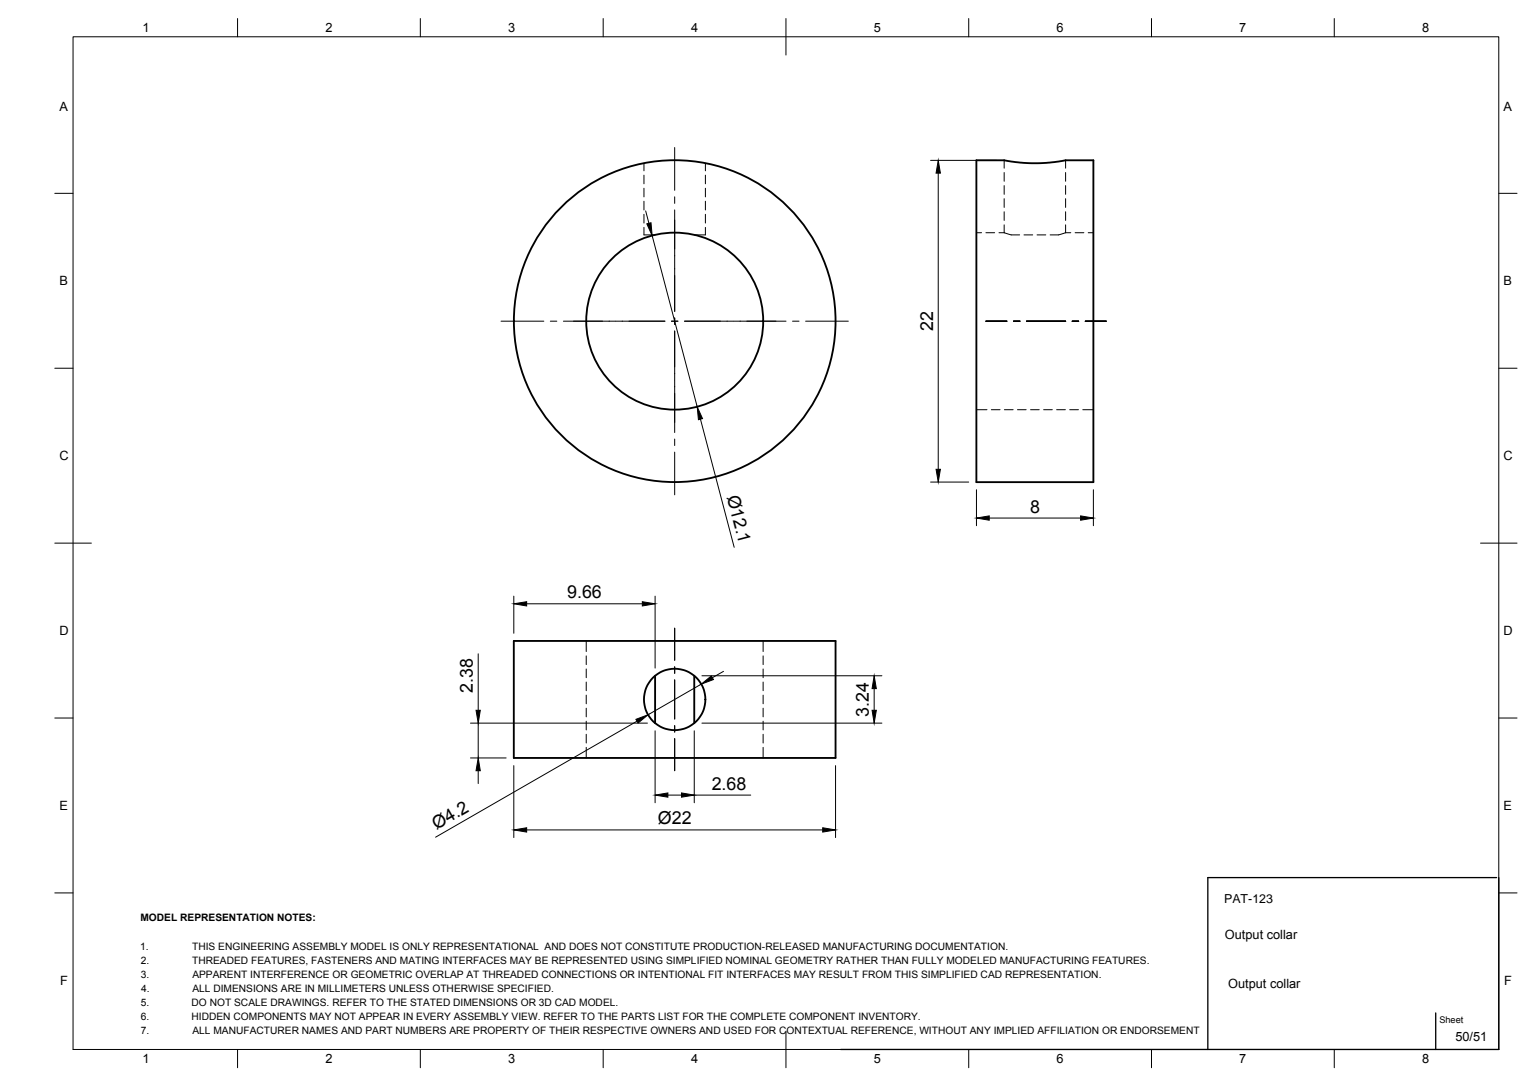
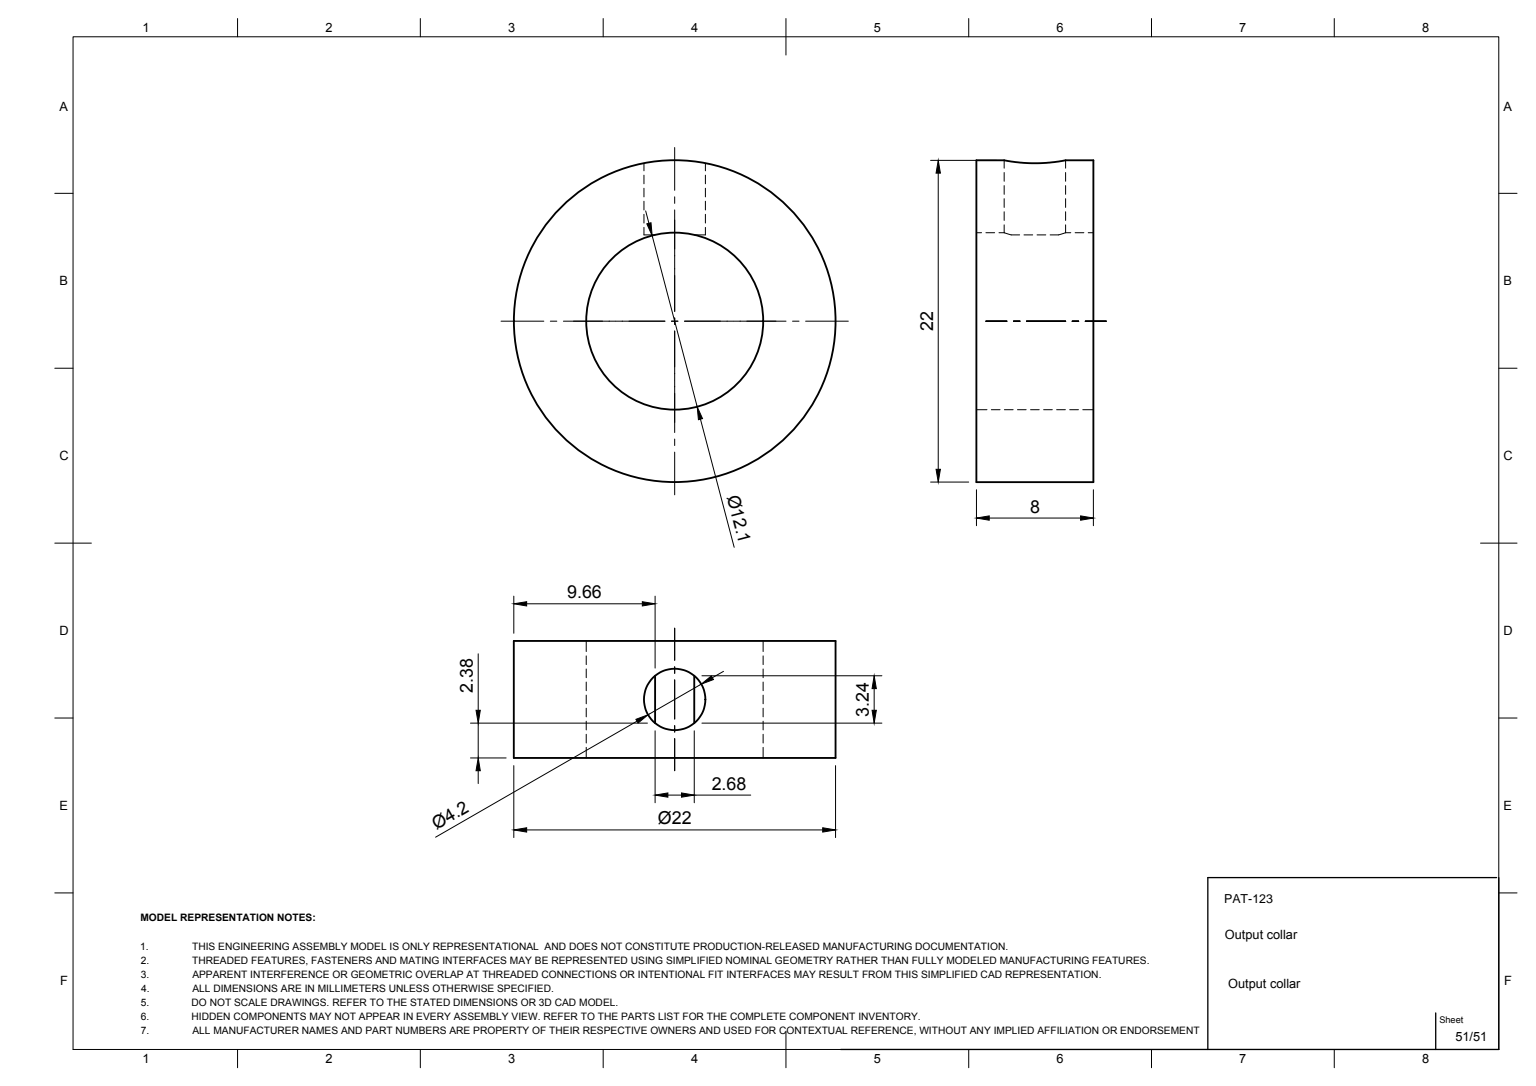
ISO-10303-21;
HEADER;
/* Generated by software containing ST-Developer
 * from STEP Tools, Inc. (www.steptools.com) 
 */

FILE_DESCRIPTION(
/* description */ ('Worm-less right-angle friction wheel drive'),
/* implementation_level */ '2;1');

FILE_NAME(
/* name */ 'Output collar.step',
/* time_stamp */ '2026-10-28T03:22:36-07:00',
/* author */ (''),
/* organization */ (''),
/* preprocessor_version */ 'ST-DEVELOPER v20.2',
/* originating_system */ 'Autodesk Translation Framework v15.17.0.0',
/* authorisation */ '');

FILE_SCHEMA (('AUTOMOTIVE_DESIGN { 1 0 10303 214 3 1 1 }'));
ENDSEC;

DATA;
#10=MECHANICAL_DESIGN_GEOMETRIC_PRESENTATION_REPRESENTATION('',(#661),#17046);
#501=B_SPLINE_CURVE_WITH_KNOTS('',3,(#16636,#16637,#16638,#16639,#16640,
#16641),.UNSPECIFIED.,.F.,.F.,(4,2,4),(0.818088904349169,0.878131747417164,
0.957937926194035),.UNSPECIFIED.);
#502=B_SPLINE_CURVE_WITH_KNOTS('',3,(#16645,#16646,#16647,#16648,#16649,
#16650),.UNSPECIFIED.,.F.,.F.,(4,2,4),(0.319312642064678,0.399118820841549,
0.459161663909543),.UNSPECIFIED.);
#503=B_SPLINE_CURVE_WITH_KNOTS('',3,(#16651,#16652,#16653,#16654,#16655,
#16656),.UNSPECIFIED.,.F.,.F.,(4,2,4),(0.179463620219813,0.239506463287807,
0.319312642064678),.UNSPECIFIED.);
#504=B_SPLINE_CURVE_WITH_KNOTS('',3,(#16657,#16658,#16659,#16660,#16661,
#16662),.UNSPECIFIED.,.F.,.F.,(4,2,4),(0.957937926194035,1.03774410497091,
1.0977869480389),.UNSPECIFIED.);
#505=B_SPLINE_CURVE_WITH_KNOTS('',3,(#16666,#16667,#16668,#16669,#16670,
#16671,#16672,#16673,#16674,#16675),.UNSPECIFIED.,.F.,.F.,(4,2,2,2,4),(0.,
0.0793157643915217,0.158631528783043,0.237943615933649,0.317255703084255),
 .UNSPECIFIED.);
#506=B_SPLINE_CURVE_WITH_KNOTS('',3,(#16677,#16678,#16679,#16680,#16681,
#16682,#16683,#16684,#16685,#16686),.UNSPECIFIED.,.F.,.F.,(4,2,2,2,4),(0.951767109252766,
1.03107919640337,1.11039128355398,1.1897070479455,1.26902281233702),
 .UNSPECIFIED.);
#507=B_SPLINE_CURVE_WITH_KNOTS('',3,(#16687,#16688,#16689,#16690,#16691,
#16692,#16693,#16694,#16695,#16696,#16697,#16698,#16699,#16700,#16701,#16702,
#16703,#16704),.UNSPECIFIED.,.F.,.F.,(4,2,2,2,2,2,2,2,4),(0.317255703084255,
0.396567790234861,0.475879877385467,0.555195641776989,0.63451140616851,
0.713827170560032,0.793142934951554,0.87245502210216,0.951767109252766),
 .UNSPECIFIED.);
#560=SHAPE_REPRESENTATION_RELATIONSHIP('SRR','None',#17306,#607);
#607=ADVANCED_BREP_SHAPE_REPRESENTATION('',(#711),#17042);
#661=STYLED_ITEM('',(#17605),#711);
#711=MANIFOLD_SOLID_BREP('Body1',#8220);
#947=FACE_BOUND('',#2343,.T.);
#948=FACE_BOUND('',#2345,.T.);
#1181=PLANE('',#9699);
#1182=PLANE('',#9703);
#1183=PLANE('',#9710);
#1184=PLANE('',#9711);
#1639=FACE_OUTER_BOUND('',#2337,.T.);
#1640=FACE_OUTER_BOUND('',#2338,.T.);
#1641=FACE_OUTER_BOUND('',#2339,.T.);
#1642=FACE_OUTER_BOUND('',#2340,.T.);
#1643=FACE_OUTER_BOUND('',#2341,.T.);
#1644=FACE_OUTER_BOUND('',#2342,.T.);
#1645=FACE_OUTER_BOUND('',#2344,.T.);
#2337=EDGE_LOOP('',(#7356,#7357));
#2338=EDGE_LOOP('',(#7358,#7359,#7360,#7361,#7362,#7363,#7364,#7365,#7366,
#7367,#7368));
#2339=EDGE_LOOP('',(#7369,#7370));
#2340=EDGE_LOOP('',(#7371,#7372,#7373,#7374,#7375,#7376,#7377,#7378,#7379,
#7380,#7381,#7382));
#2341=EDGE_LOOP('',(#7383,#7384,#7385,#7386,#7387,#7388,#7389,#7390,#7391));
#2342=EDGE_LOOP('',(#7392));
#2343=EDGE_LOOP('',(#7393));
#2344=EDGE_LOOP('',(#7394));
#2345=EDGE_LOOP('',(#7395));
#2859=LINE('',#16631,#3399);
#2860=LINE('',#16664,#3400);
#2861=LINE('',#16706,#3401);
#2862=LINE('',#16710,#3402);
#2863=LINE('',#16712,#3403);
#2864=LINE('',#16717,#3404);
#2865=LINE('',#16719,#3405);
#3399=VECTOR('',#12171,1.);
#3400=VECTOR('',#12178,0.21);
#3401=VECTOR('',#12181,1.);
#3402=VECTOR('',#12186,0.605);
#3403=VECTOR('',#12187,0.605);
#3404=VECTOR('',#12194,1.1);
#3405=VECTOR('',#12195,1.1);
#3854=CIRCLE('',#9700,0.21);
#3855=CIRCLE('',#9702,0.21);
#3856=CIRCLE('',#9705,0.605);
#3857=CIRCLE('',#9706,0.605);
#3858=CIRCLE('',#9708,1.1);
#3859=CIRCLE('',#9709,1.1);
#4479=VERTEX_POINT('',#16629);
#4480=VERTEX_POINT('',#16630);
#4481=VERTEX_POINT('',#16634);
#4482=VERTEX_POINT('',#16635);
#4483=VERTEX_POINT('',#16642);
#4484=VERTEX_POINT('',#16644);
#4485=VERTEX_POINT('',#16663);
#4486=VERTEX_POINT('',#16665);
#4487=VERTEX_POINT('',#16676);
#4488=VERTEX_POINT('',#16708);
#4489=VERTEX_POINT('',#16711);
#4490=VERTEX_POINT('',#16715);
#4491=VERTEX_POINT('',#16718);
#5447=EDGE_CURVE('',#4479,#4480,#2859,.T.);
#5448=EDGE_CURVE('',#4479,#4480,#3854,.T.);
#5449=EDGE_CURVE('',#4481,#4482,#501,.T.);
#5450=EDGE_CURVE('',#4483,#4481,#3855,.T.);
#5451=EDGE_CURVE('',#4484,#4483,#502,.T.);
#5452=EDGE_CURVE('',#4480,#4484,#503,.T.);
#5453=EDGE_CURVE('',#4482,#4479,#504,.T.);
#5454=EDGE_CURVE('',#4482,#4485,#2860,.T.);
#5455=EDGE_CURVE('',#4486,#4485,#505,.T.);
#5456=EDGE_CURVE('',#4487,#4486,#506,.T.);
#5457=EDGE_CURVE('',#4485,#4487,#507,.T.);
#5458=EDGE_CURVE('',#4483,#4481,#2861,.T.);
#5459=EDGE_CURVE('',#4488,#4488,#3856,.T.);
#5460=EDGE_CURVE('',#4488,#4484,#2862,.T.);
#5461=EDGE_CURVE('',#4482,#4489,#2863,.T.);
#5462=EDGE_CURVE('',#4489,#4489,#3857,.T.);
#5463=EDGE_CURVE('',#4490,#4490,#3858,.T.);
#5464=EDGE_CURVE('',#4490,#4487,#2864,.T.);
#5465=EDGE_CURVE('',#4485,#4491,#2865,.T.);
#5466=EDGE_CURVE('',#4491,#4491,#3859,.T.);
#7356=ORIENTED_EDGE('',*,*,#5447,.F.);
#7357=ORIENTED_EDGE('',*,*,#5448,.T.);
#7358=ORIENTED_EDGE('',*,*,#5449,.F.);
#7359=ORIENTED_EDGE('',*,*,#5450,.F.);
#7360=ORIENTED_EDGE('',*,*,#5451,.F.);
#7361=ORIENTED_EDGE('',*,*,#5452,.F.);
#7362=ORIENTED_EDGE('',*,*,#5448,.F.);
#7363=ORIENTED_EDGE('',*,*,#5453,.F.);
#7364=ORIENTED_EDGE('',*,*,#5454,.T.);
#7365=ORIENTED_EDGE('',*,*,#5455,.F.);
#7366=ORIENTED_EDGE('',*,*,#5456,.F.);
#7367=ORIENTED_EDGE('',*,*,#5457,.F.);
#7368=ORIENTED_EDGE('',*,*,#5454,.F.);
#7369=ORIENTED_EDGE('',*,*,#5458,.F.);
#7370=ORIENTED_EDGE('',*,*,#5450,.T.);
#7371=ORIENTED_EDGE('',*,*,#5459,.F.);
#7372=ORIENTED_EDGE('',*,*,#5460,.T.);
#7373=ORIENTED_EDGE('',*,*,#5451,.T.);
#7374=ORIENTED_EDGE('',*,*,#5458,.T.);
#7375=ORIENTED_EDGE('',*,*,#5449,.T.);
#7376=ORIENTED_EDGE('',*,*,#5461,.T.);
#7377=ORIENTED_EDGE('',*,*,#5462,.T.);
#7378=ORIENTED_EDGE('',*,*,#5461,.F.);
#7379=ORIENTED_EDGE('',*,*,#5453,.T.);
#7380=ORIENTED_EDGE('',*,*,#5447,.T.);
#7381=ORIENTED_EDGE('',*,*,#5452,.T.);
#7382=ORIENTED_EDGE('',*,*,#5460,.F.);
#7383=ORIENTED_EDGE('',*,*,#5463,.F.);
#7384=ORIENTED_EDGE('',*,*,#5464,.T.);
#7385=ORIENTED_EDGE('',*,*,#5456,.T.);
#7386=ORIENTED_EDGE('',*,*,#5455,.T.);
#7387=ORIENTED_EDGE('',*,*,#5465,.T.);
#7388=ORIENTED_EDGE('',*,*,#5466,.T.);
#7389=ORIENTED_EDGE('',*,*,#5465,.F.);
#7390=ORIENTED_EDGE('',*,*,#5457,.T.);
#7391=ORIENTED_EDGE('',*,*,#5464,.F.);
#7392=ORIENTED_EDGE('',*,*,#5463,.T.);
#7393=ORIENTED_EDGE('',*,*,#5459,.T.);
#7394=ORIENTED_EDGE('',*,*,#5466,.F.);
#7395=ORIENTED_EDGE('',*,*,#5462,.F.);
#7693=CYLINDRICAL_SURFACE('',#9701,0.21);
#7694=CYLINDRICAL_SURFACE('',#9704,0.605);
#7695=CYLINDRICAL_SURFACE('',#9707,1.1);
#8131=ADVANCED_FACE('',(#1639),#1181,.T.);
#8132=ADVANCED_FACE('',(#1640),#7693,.F.);
#8133=ADVANCED_FACE('',(#1641),#1182,.T.);
#8134=ADVANCED_FACE('',(#1642),#7694,.F.);
#8135=ADVANCED_FACE('',(#1643),#7695,.T.);
#8136=ADVANCED_FACE('',(#1644,#947),#1183,.T.);
#8137=ADVANCED_FACE('',(#1645,#948),#1184,.F.);
#8220=CLOSED_SHELL('',(#8131,#8132,#8133,#8134,#8135,#8136,#8137));
#9698=AXIS2_PLACEMENT_3D('',#16627,#12167,#12168);
#9699=AXIS2_PLACEMENT_3D('',#16628,#12169,#12170);
#9700=AXIS2_PLACEMENT_3D('',#16632,#12172,#12173);
#9701=AXIS2_PLACEMENT_3D('',#16633,#12174,#12175);
#9702=AXIS2_PLACEMENT_3D('',#16643,#12176,#12177);
#9703=AXIS2_PLACEMENT_3D('',#16705,#12179,#12180);
#9704=AXIS2_PLACEMENT_3D('',#16707,#12182,#12183);
#9705=AXIS2_PLACEMENT_3D('',#16709,#12184,#12185);
#9706=AXIS2_PLACEMENT_3D('',#16713,#12188,#12189);
#9707=AXIS2_PLACEMENT_3D('',#16714,#12190,#12191);
#9708=AXIS2_PLACEMENT_3D('',#16716,#12192,#12193);
#9709=AXIS2_PLACEMENT_3D('',#16720,#12196,#12197);
#9710=AXIS2_PLACEMENT_3D('',#16721,#12198,#12199);
#9711=AXIS2_PLACEMENT_3D('',#16722,#12200,#12201);
#12167=DIRECTION('axis',(0.,0.,1.));
#12168=DIRECTION('refdir',(1.,0.,0.));
#12169=DIRECTION('center_axis',(0.,0.,1.));
#12170=DIRECTION('ref_axis',(1.,0.,0.));
#12171=DIRECTION('',(1.,0.,0.));
#12172=DIRECTION('center_axis',(0.,0.,1.));
#12173=DIRECTION('ref_axis',(1.,0.,0.));
#12174=DIRECTION('center_axis',(0.,0.,1.));
#12175=DIRECTION('ref_axis',(1.,0.,0.));
#12176=DIRECTION('center_axis',(0.,0.,1.));
#12177=DIRECTION('ref_axis',(1.,0.,0.));
#12178=DIRECTION('',(0.,0.,1.));
#12179=DIRECTION('center_axis',(0.,0.,1.));
#12180=DIRECTION('ref_axis',(1.,0.,0.));
#12181=DIRECTION('',(-1.,0.,0.));
#12182=DIRECTION('center_axis',(1.,0.,0.));
#12183=DIRECTION('ref_axis',(0.,0.,-1.));
#12184=DIRECTION('center_axis',(-1.,0.,0.));
#12185=DIRECTION('ref_axis',(0.,0.,-1.));
#12186=DIRECTION('',(-1.,0.,0.));
#12187=DIRECTION('',(-1.,0.,0.));
#12188=DIRECTION('center_axis',(-1.,0.,0.));
#12189=DIRECTION('ref_axis',(0.,0.,-1.));
#12190=DIRECTION('center_axis',(1.,0.,0.));
#12191=DIRECTION('ref_axis',(0.,0.,-1.));
#12192=DIRECTION('center_axis',(1.,0.,0.));
#12193=DIRECTION('ref_axis',(0.,0.,-1.));
#12194=DIRECTION('',(-1.,0.,0.));
#12195=DIRECTION('',(-1.,0.,0.));
#12196=DIRECTION('center_axis',(1.,0.,0.));
#12197=DIRECTION('ref_axis',(0.,0.,-1.));
#12198=DIRECTION('center_axis',(1.,0.,0.));
#12199=DIRECTION('ref_axis',(0.,0.,-1.));
#12200=DIRECTION('center_axis',(1.,0.,0.));
#12201=DIRECTION('ref_axis',(0.,0.,-1.));
#16627=CARTESIAN_POINT('',(0.,0.,0.));
#16628=CARTESIAN_POINT('Origin',(-1.2,3.,7.59));
#16629=CARTESIAN_POINT('',(-1.36178689687364,2.86611572161004,7.59));
#16630=CARTESIAN_POINT('',(-1.03821310312636,2.86611572161004,7.59));
#16631=CARTESIAN_POINT('',(-1.6,2.86611572161004,7.59));
#16632=CARTESIAN_POINT('Origin',(-1.2,3.,7.59));
#16633=CARTESIAN_POINT('Origin',(-1.2,3.,7.59));
#16634=CARTESIAN_POINT('',(-1.36178689687364,3.13388427838996,7.59));
#16635=CARTESIAN_POINT('',(-1.41,3.,7.605));
#16636=CARTESIAN_POINT('Ctrl Pts',(-1.36178689687364,3.13388427838996,7.59));
#16637=CARTESIAN_POINT('Ctrl Pts',(-1.37472116821763,3.1182543952608,7.59354677224418));
#16638=CARTESIAN_POINT('Ctrl Pts',(-1.38579931658744,3.1001097876823,7.59698224789957));
#16639=CARTESIAN_POINT('Ctrl Pts',(-1.40463856105443,3.05482987213252,7.6030741628997));
#16640=CARTESIAN_POINT('Ctrl Pts',(-1.41,3.02660205959229,7.605));
#16641=CARTESIAN_POINT('Ctrl Pts',(-1.41,3.,7.605));
#16642=CARTESIAN_POINT('',(-1.03821310312636,3.13388427838996,7.59));
#16643=CARTESIAN_POINT('Origin',(-1.2,3.,7.59));
#16644=CARTESIAN_POINT('',(-0.99,3.,7.605));
#16645=CARTESIAN_POINT('Ctrl Pts',(-0.99,3.,7.605));
#16646=CARTESIAN_POINT('Ctrl Pts',(-0.99,3.02660205959229,7.605));
#16647=CARTESIAN_POINT('Ctrl Pts',(-0.995361438945571,3.05482987213252,
7.6030741628997));
#16648=CARTESIAN_POINT('Ctrl Pts',(-1.01420068341256,3.1001097876823,7.59698224789957));
#16649=CARTESIAN_POINT('Ctrl Pts',(-1.02527883178237,3.1182543952608,7.59354677224418));
#16650=CARTESIAN_POINT('Ctrl Pts',(-1.03821310312636,3.13388427838996,7.59));
#16651=CARTESIAN_POINT('Ctrl Pts',(-1.03821310312636,2.86611572161004,7.59));
#16652=CARTESIAN_POINT('Ctrl Pts',(-1.02527883178237,2.8817456047392,7.59354677224418));
#16653=CARTESIAN_POINT('Ctrl Pts',(-1.01420068341256,2.8998902123177,7.59698224789957));
#16654=CARTESIAN_POINT('Ctrl Pts',(-0.995361438945571,2.94517012786748,
7.6030741628997));
#16655=CARTESIAN_POINT('Ctrl Pts',(-0.99,2.97339794040771,7.605));
#16656=CARTESIAN_POINT('Ctrl Pts',(-0.99,3.,7.605));
#16657=CARTESIAN_POINT('Ctrl Pts',(-1.41,3.,7.605));
#16658=CARTESIAN_POINT('Ctrl Pts',(-1.41,2.97339794040771,7.605));
#16659=CARTESIAN_POINT('Ctrl Pts',(-1.40463856105443,2.94517012786748,7.6030741628997));
#16660=CARTESIAN_POINT('Ctrl Pts',(-1.38579931658744,2.8998902123177,7.59698224789957));
#16661=CARTESIAN_POINT('Ctrl Pts',(-1.37472116821763,2.8817456047392,7.59354677224418));
#16662=CARTESIAN_POINT('Ctrl Pts',(-1.36178689687364,2.86611572161004,7.59));
#16663=CARTESIAN_POINT('',(-1.41,3.,8.1));
#16664=CARTESIAN_POINT('',(-1.41,3.,7.59));
#16665=CARTESIAN_POINT('',(-1.2,2.79,8.07976849370594));
#16666=CARTESIAN_POINT('Ctrl Pts',(-1.2,2.79,8.07976849370594));
#16667=CARTESIAN_POINT('Ctrl Pts',(-1.22643858813051,2.79,8.07976849370594));
#16668=CARTESIAN_POINT('Ctrl Pts',(-1.25459378125493,2.79529707732902,8.08084015664674));
#16669=CARTESIAN_POINT('Ctrl Pts',(-1.30631344554134,2.81674820319365,8.08468313707126));
#16670=CARTESIAN_POINT('Ctrl Pts',(-1.32988367074114,2.83289882264279,8.08739593054622));
#16671=CARTESIAN_POINT('Ctrl Pts',(-1.36710031461738,2.87011546651904,8.09246633289124));
#16672=CARTESIAN_POINT('Ctrl Pts',(-1.38325161016341,2.89368605924271,8.09515738895358));
#16673=CARTESIAN_POINT('Ctrl Pts',(-1.40470322656974,2.94540699667048,8.09895039220591));
#16674=CARTESIAN_POINT('Ctrl Pts',(-1.41,2.97356263761646,8.1));
#16675=CARTESIAN_POINT('Ctrl Pts',(-1.41,3.,8.1));
#16676=CARTESIAN_POINT('',(-0.99,3.,8.1));
#16677=CARTESIAN_POINT('Ctrl Pts',(-0.99,3.,8.1));
#16678=CARTESIAN_POINT('Ctrl Pts',(-0.99,2.97356263761646,8.1));
#16679=CARTESIAN_POINT('Ctrl Pts',(-0.995296773430262,2.94540699667048,
8.09895039220591));
#16680=CARTESIAN_POINT('Ctrl Pts',(-1.01674838983659,2.89368605924271,8.09515738895358));
#16681=CARTESIAN_POINT('Ctrl Pts',(-1.03289968538261,2.87011546651904,8.09246633289124));
#16682=CARTESIAN_POINT('Ctrl Pts',(-1.07011632925886,2.83289882264279,8.08739593054622));
#16683=CARTESIAN_POINT('Ctrl Pts',(-1.09368655445866,2.81674820319365,8.08468313707126));
#16684=CARTESIAN_POINT('Ctrl Pts',(-1.14540621874507,2.79529707732902,8.08084015664674));
#16685=CARTESIAN_POINT('Ctrl Pts',(-1.17356141186949,2.79,8.07976849370594));
#16686=CARTESIAN_POINT('Ctrl Pts',(-1.2,2.79,8.07976849370594));
#16687=CARTESIAN_POINT('Ctrl Pts',(-1.41,3.,8.1));
#16688=CARTESIAN_POINT('Ctrl Pts',(-1.41,3.02643736238354,8.1));
#16689=CARTESIAN_POINT('Ctrl Pts',(-1.40470322656974,3.05459300332952,8.09895039220591));
#16690=CARTESIAN_POINT('Ctrl Pts',(-1.38325161016341,3.10631394075729,8.09515738895358));
#16691=CARTESIAN_POINT('Ctrl Pts',(-1.36710031461738,3.12988453348096,8.09246633289124));
#16692=CARTESIAN_POINT('Ctrl Pts',(-1.32988367074114,3.16710117735721,8.08739593054622));
#16693=CARTESIAN_POINT('Ctrl Pts',(-1.30631344554134,3.18325179680635,8.08468313707126));
#16694=CARTESIAN_POINT('Ctrl Pts',(-1.25459378125493,3.20470292267098,8.08084015664674));
#16695=CARTESIAN_POINT('Ctrl Pts',(-1.22643858813051,3.21,8.07976849370594));
#16696=CARTESIAN_POINT('Ctrl Pts',(-1.17356141186949,3.21,8.07976849370594));
#16697=CARTESIAN_POINT('Ctrl Pts',(-1.14540621874507,3.20470292267098,8.08084015664674));
#16698=CARTESIAN_POINT('Ctrl Pts',(-1.09368655445866,3.18325179680635,8.08468313707126));
#16699=CARTESIAN_POINT('Ctrl Pts',(-1.07011632925886,3.16710117735721,8.08739593054622));
#16700=CARTESIAN_POINT('Ctrl Pts',(-1.03289968538262,3.12988453348096,8.09246633289124));
#16701=CARTESIAN_POINT('Ctrl Pts',(-1.01674838983659,3.10631394075729,8.09515738895358));
#16702=CARTESIAN_POINT('Ctrl Pts',(-0.995296773430262,3.05459300332952,
8.09895039220591));
#16703=CARTESIAN_POINT('Ctrl Pts',(-0.99,3.02643736238354,8.1));
#16704=CARTESIAN_POINT('Ctrl Pts',(-0.99,3.,8.1));
#16705=CARTESIAN_POINT('Origin',(-1.2,3.,7.59));
#16706=CARTESIAN_POINT('',(-1.6,3.13388427838996,7.59));
#16707=CARTESIAN_POINT('Origin',(-1.6,3.,7.));
#16708=CARTESIAN_POINT('',(-0.8,3.,7.605));
#16709=CARTESIAN_POINT('Origin',(-0.8,3.,7.));
#16710=CARTESIAN_POINT('',(-1.6,3.,7.605));
#16711=CARTESIAN_POINT('',(-1.6,3.,7.605));
#16712=CARTESIAN_POINT('',(-1.6,3.,7.605));
#16713=CARTESIAN_POINT('Origin',(-1.6,3.,7.));
#16714=CARTESIAN_POINT('Origin',(-1.6,3.,7.));
#16715=CARTESIAN_POINT('',(-0.8,3.,8.1));
#16716=CARTESIAN_POINT('Origin',(-0.8,3.,7.));
#16717=CARTESIAN_POINT('',(-1.6,3.,8.1));
#16718=CARTESIAN_POINT('',(-1.6,3.,8.1));
#16719=CARTESIAN_POINT('',(-1.6,3.,8.1));
#16720=CARTESIAN_POINT('Origin',(-1.6,3.,7.));
#16721=CARTESIAN_POINT('Origin',(-0.8,3.,7.));
#16722=CARTESIAN_POINT('Origin',(-1.6,3.,7.));
#16989=UNCERTAINTY_MEASURE_WITH_UNIT(LENGTH_MEASURE(0.001),#17047,
'DISTANCE_ACCURACY_VALUE',
'Maximum model space distance between geometric entities at asserted c
onnectivities');
#16993=UNCERTAINTY_MEASURE_WITH_UNIT(LENGTH_MEASURE(0.001),#17047,
'DISTANCE_ACCURACY_VALUE',
'Maximum model space distance between geometric entities at asserted c
onnectivities');
#17042=(
GEOMETRIC_REPRESENTATION_CONTEXT(3)
GLOBAL_UNCERTAINTY_ASSIGNED_CONTEXT((#16989))
GLOBAL_UNIT_ASSIGNED_CONTEXT((#17047,#17049,#17050))
REPRESENTATION_CONTEXT('','3D')
);
#17046=(
GEOMETRIC_REPRESENTATION_CONTEXT(3)
GLOBAL_UNCERTAINTY_ASSIGNED_CONTEXT((#16993))
GLOBAL_UNIT_ASSIGNED_CONTEXT((#17047,#17049,#17050))
REPRESENTATION_CONTEXT('','3D')
);
#17047=(
LENGTH_UNIT()
NAMED_UNIT(*)
SI_UNIT(.CENTI.,.METRE.)
);
#17049=(
NAMED_UNIT(*)
PLANE_ANGLE_UNIT()
SI_UNIT($,.RADIAN.)
);
#17050=(
NAMED_UNIT(*)
SI_UNIT($,.STERADIAN.)
SOLID_ANGLE_UNIT()
);
#17099=SHAPE_DEFINITION_REPRESENTATION(#17233,#17306);
#17233=PRODUCT_DEFINITION_SHAPE('',$,#17359);
#17306=SHAPE_REPRESENTATION('',(#9698),#17042);
#17310=PRODUCT_DEFINITION_CONTEXT('part definition',#17468,'design');
#17359=PRODUCT_DEFINITION('Output collar','Output collar',#17411,#17310);
#17411=PRODUCT_DEFINITION_FORMATION('',$,#17518);
#17468=APPLICATION_CONTEXT(
'Core Data for Automotive Mechanical Design Process');
#17469=PRODUCT_CONTEXT('part definition',#17468,'mechanical');
#17518=PRODUCT('Output collar','Output collar','Output collar',(#17469));
#17599=COLOUR_RGB('Off White',0.89,0.88,0.83);
#17600=FILL_AREA_STYLE_COLOUR('',#17599);
#17601=FILL_AREA_STYLE('',(#17600));
#17602=SURFACE_STYLE_FILL_AREA(#17601);
#17603=SURFACE_SIDE_STYLE('',(#17602));
#17604=SURFACE_STYLE_USAGE(.BOTH.,#17603);
#17605=PRESENTATION_STYLE_ASSIGNMENT((#17604));
ENDSEC;
END-ISO-10303-21;
